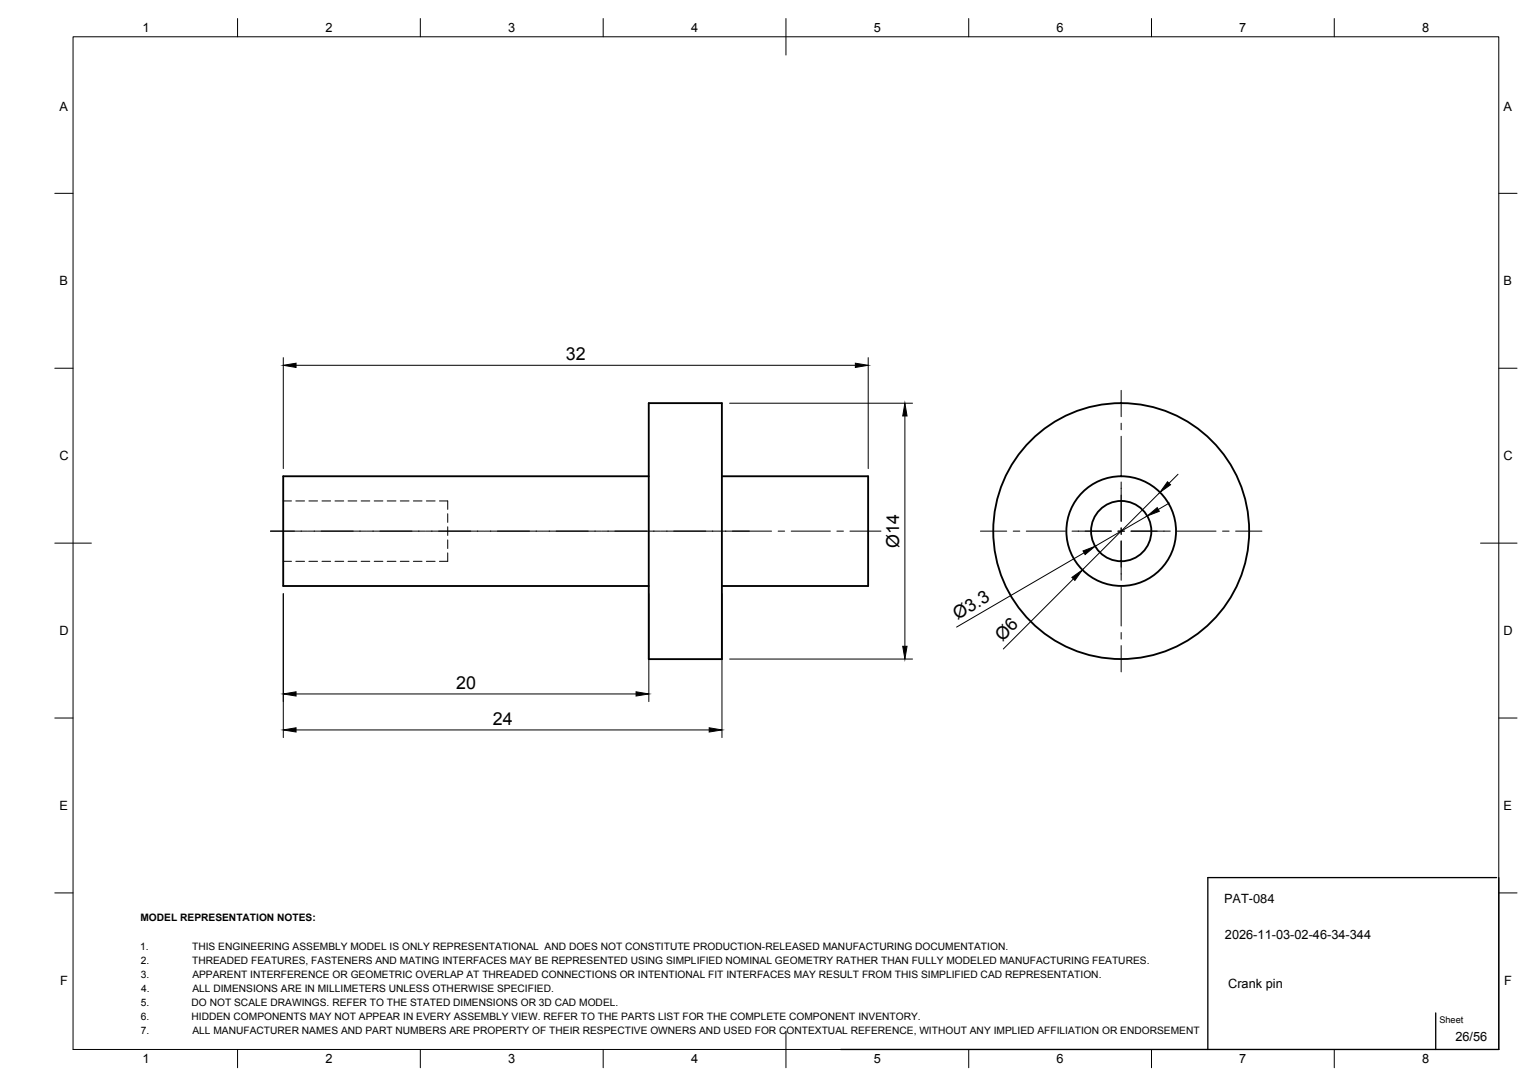
ISO-10303-21;
HEADER;
/* Generated by software containing ST-Developer
 * from STEP Tools, Inc. (www.steptools.com) 
 */

FILE_DESCRIPTION(
/* description */ ('Quick-return (Whitworth) mechanism'),
/* implementation_level */ '2;1');

FILE_NAME(
/* name */ 'Crank pin.step',
/* time_stamp */ '2026-10-28T03:25:57-07:00',
/* author */ (''),
/* organization */ (''),
/* preprocessor_version */ 'ST-DEVELOPER v20.2',
/* originating_system */ 'Autodesk Translation Framework v15.17.0.0',
/* authorisation */ '');

FILE_SCHEMA (('AUTOMOTIVE_DESIGN { 1 0 10303 214 3 1 1 }'));
ENDSEC;

DATA;
#10=MECHANICAL_DESIGN_GEOMETRIC_PRESENTATION_REPRESENTATION('',(#515),#14878);
#419=SHAPE_REPRESENTATION_RELATIONSHIP('SRR','None',#15089,#463);
#463=ADVANCED_BREP_SHAPE_REPRESENTATION('',(#567),#14846);
#515=STYLED_ITEM('',(#15406),#567);
#567=MANIFOLD_SOLID_BREP('Body1',#7869);
#715=FACE_BOUND('',#1873,.T.);
#716=FACE_BOUND('',#1875,.T.);
#717=FACE_BOUND('',#1880,.T.);
#890=PLANE('',#8913);
#891=PLANE('',#8914);
#892=PLANE('',#8917);
#893=PLANE('',#8925);
#894=PLANE('',#8926);
#1280=FACE_OUTER_BOUND('',#1870,.T.);
#1281=FACE_OUTER_BOUND('',#1871,.T.);
#1282=FACE_OUTER_BOUND('',#1872,.T.);
#1283=FACE_OUTER_BOUND('',#1874,.T.);
#1284=FACE_OUTER_BOUND('',#1876,.T.);
#1285=FACE_OUTER_BOUND('',#1877,.T.);
#1286=FACE_OUTER_BOUND('',#1878,.T.);
#1287=FACE_OUTER_BOUND('',#1879,.T.);
#1288=FACE_OUTER_BOUND('',#1881,.T.);
#1870=EDGE_LOOP('',(#6258,#6259,#6260,#6261));
#1871=EDGE_LOOP('',(#6262));
#1872=EDGE_LOOP('',(#6263));
#1873=EDGE_LOOP('',(#6264));
#1874=EDGE_LOOP('',(#6265));
#1875=EDGE_LOOP('',(#6266));
#1876=EDGE_LOOP('',(#6267,#6268,#6269,#6270));
#1877=EDGE_LOOP('',(#6271,#6272,#6273,#6274));
#1878=EDGE_LOOP('',(#6275,#6276,#6277,#6278));
#1879=EDGE_LOOP('',(#6279));
#1880=EDGE_LOOP('',(#6280));
#1881=EDGE_LOOP('',(#6281));
#2371=LINE('',#13586,#2894);
#2372=LINE('',#13600,#2895);
#2373=LINE('',#13603,#2896);
#2374=LINE('',#13608,#2897);
#2894=VECTOR('',#10654,0.165);
#2895=VECTOR('',#10673,0.7);
#2896=VECTOR('',#10676,0.3);
#2897=VECTOR('',#10683,0.3);
#3482=CIRCLE('',#8911,0.165);
#3483=CIRCLE('',#8912,0.165);
#3484=CIRCLE('',#8915,0.7);
#3485=CIRCLE('',#8916,0.3);
#3486=CIRCLE('',#8918,0.7);
#3487=CIRCLE('',#8919,0.3);
#3488=CIRCLE('',#8922,0.3);
#3489=CIRCLE('',#8924,0.3);
#3974=VERTEX_POINT('',#13583);
#3975=VERTEX_POINT('',#13585);
#3976=VERTEX_POINT('',#13590);
#3977=VERTEX_POINT('',#13592);
#3978=VERTEX_POINT('',#13595);
#3979=VERTEX_POINT('',#13597);
#3980=VERTEX_POINT('',#13602);
#3981=VERTEX_POINT('',#13606);
#4786=EDGE_CURVE('',#3974,#3974,#3482,.T.);
#4787=EDGE_CURVE('',#3974,#3975,#2371,.T.);
#4788=EDGE_CURVE('',#3975,#3975,#3483,.T.);
#4789=EDGE_CURVE('',#3976,#3976,#3484,.T.);
#4790=EDGE_CURVE('',#3977,#3977,#3485,.T.);
#4791=EDGE_CURVE('',#3978,#3978,#3486,.T.);
#4792=EDGE_CURVE('',#3979,#3979,#3487,.T.);
#4793=EDGE_CURVE('',#3976,#3978,#2372,.T.);
#4794=EDGE_CURVE('',#3979,#3980,#2373,.T.);
#4795=EDGE_CURVE('',#3980,#3980,#3488,.T.);
#4796=EDGE_CURVE('',#3981,#3981,#3489,.T.);
#4797=EDGE_CURVE('',#3981,#3977,#2374,.T.);
#6258=ORIENTED_EDGE('',*,*,#4786,.F.);
#6259=ORIENTED_EDGE('',*,*,#4787,.T.);
#6260=ORIENTED_EDGE('',*,*,#4788,.F.);
#6261=ORIENTED_EDGE('',*,*,#4787,.F.);
#6262=ORIENTED_EDGE('',*,*,#4786,.T.);
#6263=ORIENTED_EDGE('',*,*,#4789,.T.);
#6264=ORIENTED_EDGE('',*,*,#4790,.F.);
#6265=ORIENTED_EDGE('',*,*,#4791,.F.);
#6266=ORIENTED_EDGE('',*,*,#4792,.F.);
#6267=ORIENTED_EDGE('',*,*,#4789,.F.);
#6268=ORIENTED_EDGE('',*,*,#4793,.T.);
#6269=ORIENTED_EDGE('',*,*,#4791,.T.);
#6270=ORIENTED_EDGE('',*,*,#4793,.F.);
#6271=ORIENTED_EDGE('',*,*,#4792,.T.);
#6272=ORIENTED_EDGE('',*,*,#4794,.T.);
#6273=ORIENTED_EDGE('',*,*,#4795,.T.);
#6274=ORIENTED_EDGE('',*,*,#4794,.F.);
#6275=ORIENTED_EDGE('',*,*,#4796,.F.);
#6276=ORIENTED_EDGE('',*,*,#4797,.T.);
#6277=ORIENTED_EDGE('',*,*,#4790,.T.);
#6278=ORIENTED_EDGE('',*,*,#4797,.F.);
#6279=ORIENTED_EDGE('',*,*,#4796,.T.);
#6280=ORIENTED_EDGE('',*,*,#4788,.T.);
#6281=ORIENTED_EDGE('',*,*,#4795,.F.);
#7313=CYLINDRICAL_SURFACE('',#8910,0.165);
#7314=CYLINDRICAL_SURFACE('',#8920,0.7);
#7315=CYLINDRICAL_SURFACE('',#8921,0.3);
#7316=CYLINDRICAL_SURFACE('',#8923,0.3);
#7611=ADVANCED_FACE('',(#1280),#7313,.F.);
#7612=ADVANCED_FACE('',(#1281),#890,.T.);
#7613=ADVANCED_FACE('',(#1282,#715),#891,.T.);
#7614=ADVANCED_FACE('',(#1283,#716),#892,.F.);
#7615=ADVANCED_FACE('',(#1284),#7314,.T.);
#7616=ADVANCED_FACE('',(#1285),#7315,.T.);
#7617=ADVANCED_FACE('',(#1286),#7316,.T.);
#7618=ADVANCED_FACE('',(#1287,#717),#893,.T.);
#7619=ADVANCED_FACE('',(#1288),#894,.F.);
#7869=CLOSED_SHELL('',(#7611,#7612,#7613,#7614,#7615,#7616,#7617,#7618,
#7619));
#8909=AXIS2_PLACEMENT_3D('',#13581,#10648,#10649);
#8910=AXIS2_PLACEMENT_3D('',#13582,#10650,#10651);
#8911=AXIS2_PLACEMENT_3D('',#13584,#10652,#10653);
#8912=AXIS2_PLACEMENT_3D('',#13587,#10655,#10656);
#8913=AXIS2_PLACEMENT_3D('',#13588,#10657,#10658);
#8914=AXIS2_PLACEMENT_3D('',#13589,#10659,#10660);
#8915=AXIS2_PLACEMENT_3D('',#13591,#10661,#10662);
#8916=AXIS2_PLACEMENT_3D('',#13593,#10663,#10664);
#8917=AXIS2_PLACEMENT_3D('',#13594,#10665,#10666);
#8918=AXIS2_PLACEMENT_3D('',#13596,#10667,#10668);
#8919=AXIS2_PLACEMENT_3D('',#13598,#10669,#10670);
#8920=AXIS2_PLACEMENT_3D('',#13599,#10671,#10672);
#8921=AXIS2_PLACEMENT_3D('',#13601,#10674,#10675);
#8922=AXIS2_PLACEMENT_3D('',#13604,#10677,#10678);
#8923=AXIS2_PLACEMENT_3D('',#13605,#10679,#10680);
#8924=AXIS2_PLACEMENT_3D('',#13607,#10681,#10682);
#8925=AXIS2_PLACEMENT_3D('',#13609,#10684,#10685);
#8926=AXIS2_PLACEMENT_3D('',#13610,#10686,#10687);
#10648=DIRECTION('axis',(0.,0.,1.));
#10649=DIRECTION('refdir',(1.,0.,0.));
#10650=DIRECTION('center_axis',(0.,0.,1.));
#10651=DIRECTION('ref_axis',(1.,0.,0.));
#10652=DIRECTION('center_axis',(0.,0.,1.));
#10653=DIRECTION('ref_axis',(1.,0.,0.));
#10654=DIRECTION('',(0.,0.,1.));
#10655=DIRECTION('center_axis',(0.,0.,-1.));
#10656=DIRECTION('ref_axis',(1.,0.,0.));
#10657=DIRECTION('center_axis',(0.,0.,1.));
#10658=DIRECTION('ref_axis',(1.,0.,0.));
#10659=DIRECTION('center_axis',(0.,0.,1.));
#10660=DIRECTION('ref_axis',(1.,0.,0.));
#10661=DIRECTION('center_axis',(0.,0.,1.));
#10662=DIRECTION('ref_axis',(1.,0.,0.));
#10663=DIRECTION('center_axis',(0.,0.,1.));
#10664=DIRECTION('ref_axis',(1.,0.,0.));
#10665=DIRECTION('center_axis',(0.,0.,1.));
#10666=DIRECTION('ref_axis',(1.,0.,0.));
#10667=DIRECTION('center_axis',(0.,0.,1.));
#10668=DIRECTION('ref_axis',(1.,0.,0.));
#10669=DIRECTION('center_axis',(0.,0.,-1.));
#10670=DIRECTION('ref_axis',(1.,0.,0.));
#10671=DIRECTION('center_axis',(0.,0.,1.));
#10672=DIRECTION('ref_axis',(1.,0.,0.));
#10673=DIRECTION('',(0.,0.,-1.));
#10674=DIRECTION('center_axis',(0.,0.,1.));
#10675=DIRECTION('ref_axis',(1.,0.,0.));
#10676=DIRECTION('',(0.,0.,-1.));
#10677=DIRECTION('center_axis',(0.,0.,1.));
#10678=DIRECTION('ref_axis',(1.,0.,0.));
#10679=DIRECTION('center_axis',(0.,0.,1.));
#10680=DIRECTION('ref_axis',(1.,0.,0.));
#10681=DIRECTION('center_axis',(0.,0.,1.));
#10682=DIRECTION('ref_axis',(1.,0.,0.));
#10683=DIRECTION('',(0.,0.,-1.));
#10684=DIRECTION('center_axis',(0.,0.,1.));
#10685=DIRECTION('ref_axis',(1.,0.,0.));
#10686=DIRECTION('center_axis',(0.,0.,1.));
#10687=DIRECTION('ref_axis',(1.,0.,0.));
#13581=CARTESIAN_POINT('',(0.,0.,0.));
#13582=CARTESIAN_POINT('Origin',(0.,9.,7.1));
#13583=CARTESIAN_POINT('',(-0.165,9.,7.1));
#13584=CARTESIAN_POINT('Origin',(0.,9.,7.1));
#13585=CARTESIAN_POINT('',(-0.165,9.,8.));
#13586=CARTESIAN_POINT('',(-0.165,9.,7.1));
#13587=CARTESIAN_POINT('Origin',(0.,9.,8.));
#13588=CARTESIAN_POINT('Origin',(0.,9.,7.1));
#13589=CARTESIAN_POINT('Origin',(0.,9.,6.));
#13590=CARTESIAN_POINT('',(-0.7,9.,6.));
#13591=CARTESIAN_POINT('Origin',(0.,9.,6.));
#13592=CARTESIAN_POINT('',(-0.3,9.,6.));
#13593=CARTESIAN_POINT('Origin',(0.,9.,6.));
#13594=CARTESIAN_POINT('Origin',(0.,9.,5.6));
#13595=CARTESIAN_POINT('',(-0.7,9.,5.6));
#13596=CARTESIAN_POINT('Origin',(0.,9.,5.6));
#13597=CARTESIAN_POINT('',(-0.3,9.,5.6));
#13598=CARTESIAN_POINT('Origin',(0.,9.,5.6));
#13599=CARTESIAN_POINT('Origin',(0.,9.,5.6));
#13600=CARTESIAN_POINT('',(-0.7,9.,5.6));
#13601=CARTESIAN_POINT('Origin',(0.,9.,4.8));
#13602=CARTESIAN_POINT('',(-0.3,9.,4.8));
#13603=CARTESIAN_POINT('',(-0.3,9.,4.8));
#13604=CARTESIAN_POINT('Origin',(0.,9.,4.8));
#13605=CARTESIAN_POINT('Origin',(0.,9.,4.8));
#13606=CARTESIAN_POINT('',(-0.3,9.,8.));
#13607=CARTESIAN_POINT('Origin',(0.,9.,8.));
#13608=CARTESIAN_POINT('',(-0.3,9.,4.8));
#13609=CARTESIAN_POINT('Origin',(0.,9.,8.));
#13610=CARTESIAN_POINT('Origin',(0.,9.,4.8));
#14792=UNCERTAINTY_MEASURE_WITH_UNIT(LENGTH_MEASURE(0.001),#14879,
'DISTANCE_ACCURACY_VALUE',
'Maximum model space distance between geometric entities at asserted c
onnectivities');
#14824=UNCERTAINTY_MEASURE_WITH_UNIT(LENGTH_MEASURE(0.001),#14879,
'DISTANCE_ACCURACY_VALUE',
'Maximum model space distance between geometric entities at asserted c
onnectivities');
#14846=(
GEOMETRIC_REPRESENTATION_CONTEXT(3)
GLOBAL_UNCERTAINTY_ASSIGNED_CONTEXT((#14792))
GLOBAL_UNIT_ASSIGNED_CONTEXT((#14879,#14881,#14882))
REPRESENTATION_CONTEXT('','3D')
);
#14878=(
GEOMETRIC_REPRESENTATION_CONTEXT(3)
GLOBAL_UNCERTAINTY_ASSIGNED_CONTEXT((#14824))
GLOBAL_UNIT_ASSIGNED_CONTEXT((#14879,#14881,#14882))
REPRESENTATION_CONTEXT('','3D')
);
#14879=(
LENGTH_UNIT()
NAMED_UNIT(*)
SI_UNIT(.CENTI.,.METRE.)
);
#14881=(
NAMED_UNIT(*)
PLANE_ANGLE_UNIT()
SI_UNIT($,.RADIAN.)
);
#14882=(
NAMED_UNIT(*)
SI_UNIT($,.STERADIAN.)
SOLID_ANGLE_UNIT()
);
#14904=SHAPE_DEFINITION_REPRESENTATION(#14962,#15089);
#14962=PRODUCT_DEFINITION_SHAPE('',$,#15143);
#15089=SHAPE_REPRESENTATION('',(#8909),#14846);
#15121=PRODUCT_DEFINITION_CONTEXT('part definition',#15282,'design');
#15143=PRODUCT_DEFINITION('Crank pin','Crank pin',#15196,#15121);
#15196=PRODUCT_DEFINITION_FORMATION('',$,#15305);
#15282=APPLICATION_CONTEXT(
'Core Data for Automotive Mechanical Design Process');
#15283=PRODUCT_CONTEXT('part definition',#15282,'mechanical');
#15305=PRODUCT('Crank pin','Crank pin','Crank pin',(#15283));
#15400=COLOUR_RGB('Grey',0.48,0.52,0.57);
#15401=FILL_AREA_STYLE_COLOUR('',#15400);
#15402=FILL_AREA_STYLE('',(#15401));
#15403=SURFACE_STYLE_FILL_AREA(#15402);
#15404=SURFACE_SIDE_STYLE('',(#15403));
#15405=SURFACE_STYLE_USAGE(.BOTH.,#15404);
#15406=PRESENTATION_STYLE_ASSIGNMENT((#15405));
ENDSEC;
END-ISO-10303-21;
